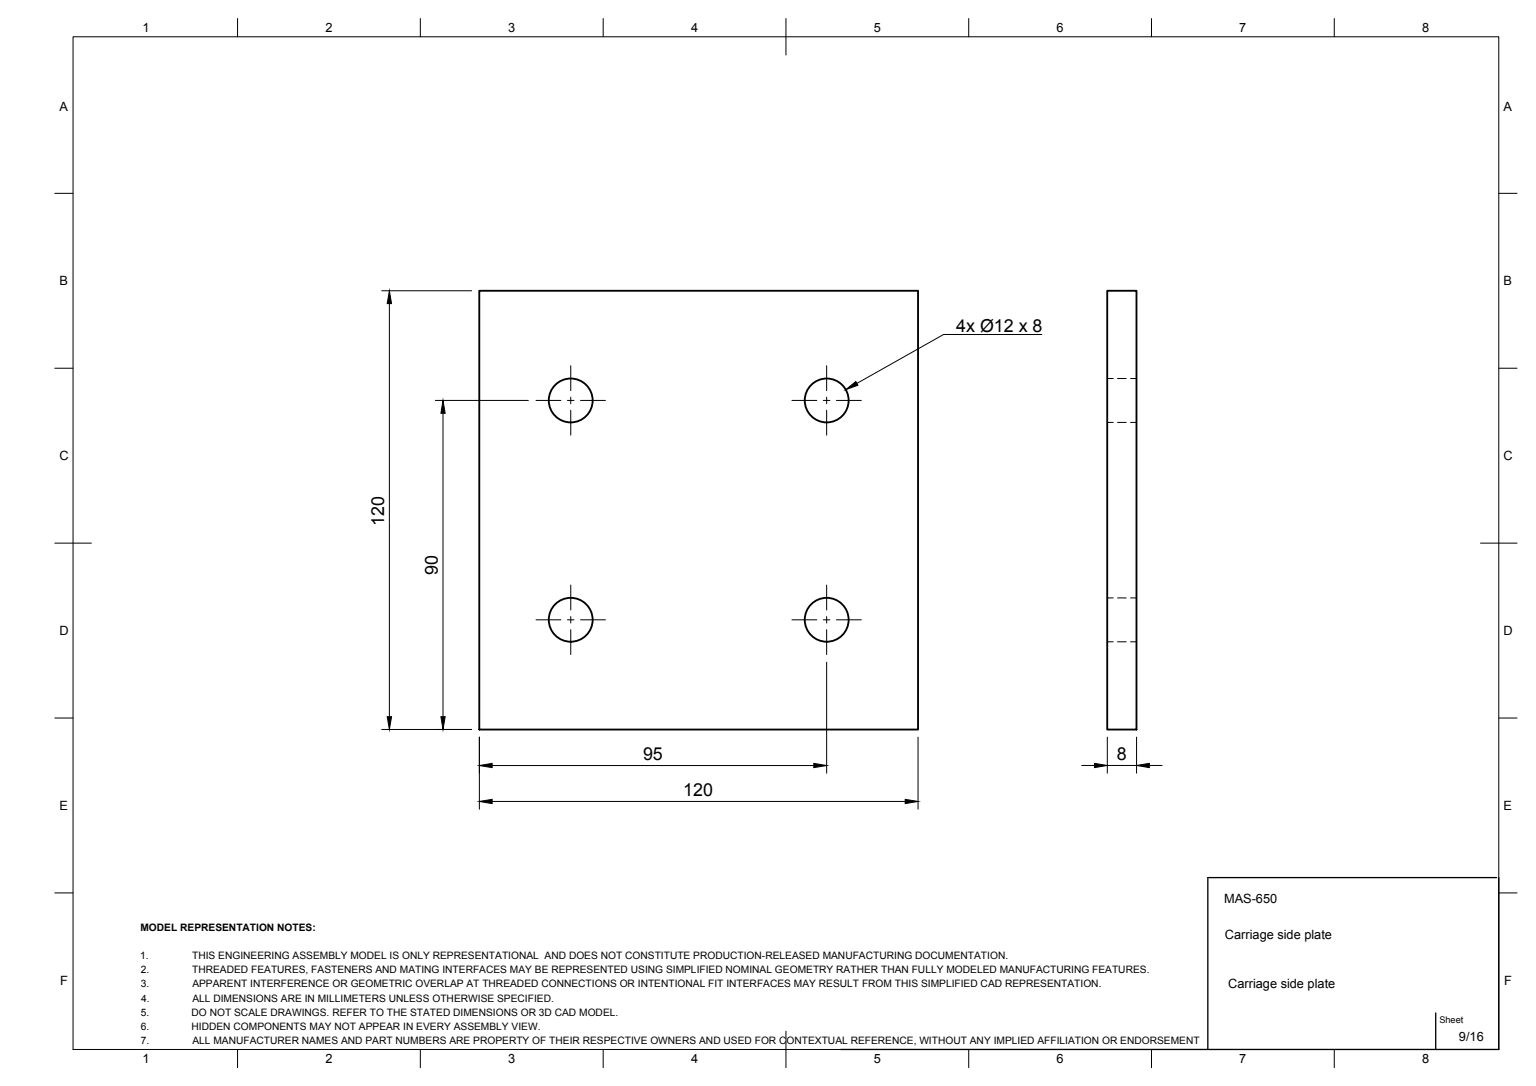
ISO-10303-21;
HEADER;
/* Generated by software containing ST-Developer
 * from STEP Tools, Inc. (www.steptools.com) 
 */

FILE_DESCRIPTION(
/* description */ ('Independent manual traversing gantry with native reusable aluminum pr
ofiles,180mm captured carriage travel, four bronze-bushed rollers, lin
ked ideal rolling motion, bonded acetal lateral guides, positive welde
d end stops and fully retained axle stacks. Editable native profile cu
t lengths220/400mm. Tool attachments viaM6 bridge-plate taps; mounted 
tool outside assembly. Welds, anchors, adhesives, fits, traction, load
/speed/structural/life ratings unassigned.'),
/* implementation_level */ '2;1');

FILE_NAME(
/* name */ 'Carriage side plate.step',
/* time_stamp */ '2026-11-09T20:04:38-08:00',
/* author */ (''),
/* organization */ (''),
/* preprocessor_version */ 'ST-DEVELOPER v20.2',
/* originating_system */ 'Autodesk Translation Framework v15.17.0.0',
/* authorisation */ '');

FILE_SCHEMA (('AUTOMOTIVE_DESIGN { 1 0 10303 214 3 1 1 }'));
ENDSEC;

DATA;
#10=MECHANICAL_DESIGN_GEOMETRIC_PRESENTATION_REPRESENTATION('',(#477),#13231);
#445=SHAPE_REPRESENTATION_RELATIONSHIP('SRR','None',#13334,#461);
#461=ADVANCED_BREP_SHAPE_REPRESENTATION('',(#493),#13221);
#477=STYLED_ITEM('',(#13423),#493);
#493=MANIFOLD_SOLID_BREP('Body1',#4157);
#523=FACE_BOUND('',#947,.T.);
#524=FACE_BOUND('',#948,.T.);
#525=FACE_BOUND('',#949,.T.);
#526=FACE_BOUND('',#950,.T.);
#527=FACE_BOUND('',#953,.T.);
#528=FACE_BOUND('',#954,.T.);
#529=FACE_BOUND('',#955,.T.);
#530=FACE_BOUND('',#956,.T.);
#596=PLANE('',#4480);
#597=PLANE('',#4481);
#598=PLANE('',#4482);
#599=PLANE('',#4483);
#600=PLANE('',#4484);
#601=PLANE('',#4485);
#701=FACE_OUTER_BOUND('',#942,.T.);
#702=FACE_OUTER_BOUND('',#943,.T.);
#703=FACE_OUTER_BOUND('',#944,.T.);
#704=FACE_OUTER_BOUND('',#945,.T.);
#705=FACE_OUTER_BOUND('',#946,.T.);
#706=FACE_OUTER_BOUND('',#951,.T.);
#707=FACE_OUTER_BOUND('',#952,.T.);
#708=FACE_OUTER_BOUND('',#957,.T.);
#709=FACE_OUTER_BOUND('',#958,.T.);
#710=FACE_OUTER_BOUND('',#959,.T.);
#942=EDGE_LOOP('',(#3018,#3019,#3020,#3021));
#943=EDGE_LOOP('',(#3022,#3023,#3024,#3025));
#944=EDGE_LOOP('',(#3026,#3027,#3028,#3029));
#945=EDGE_LOOP('',(#3030,#3031,#3032,#3033));
#946=EDGE_LOOP('',(#3034,#3035,#3036,#3037));
#947=EDGE_LOOP('',(#3038));
#948=EDGE_LOOP('',(#3039));
#949=EDGE_LOOP('',(#3040));
#950=EDGE_LOOP('',(#3041));
#951=EDGE_LOOP('',(#3042,#3043,#3044,#3045));
#952=EDGE_LOOP('',(#3046,#3047,#3048,#3049));
#953=EDGE_LOOP('',(#3050));
#954=EDGE_LOOP('',(#3051));
#955=EDGE_LOOP('',(#3052));
#956=EDGE_LOOP('',(#3053));
#957=EDGE_LOOP('',(#3054,#3055,#3056,#3057));
#958=EDGE_LOOP('',(#3058,#3059,#3060,#3061));
#959=EDGE_LOOP('',(#3062,#3063,#3064,#3065));
#1244=LINE('',#6139,#1506);
#1245=LINE('',#6145,#1507);
#1246=LINE('',#6151,#1508);
#1247=LINE('',#6157,#1509);
#1248=LINE('',#6162,#1510);
#1249=LINE('',#6164,#1511);
#1250=LINE('',#6166,#1512);
#1251=LINE('',#6167,#1513);
#1252=LINE('',#6170,#1514);
#1253=LINE('',#6172,#1515);
#1254=LINE('',#6173,#1516);
#1255=LINE('',#6176,#1517);
#1256=LINE('',#6178,#1518);
#1257=LINE('',#6179,#1519);
#1258=LINE('',#6181,#1520);
#1259=LINE('',#6182,#1521);
#1506=VECTOR('',#5107,6.);
#1507=VECTOR('',#5114,6.);
#1508=VECTOR('',#5121,6.);
#1509=VECTOR('',#5128,6.);
#1510=VECTOR('',#5133,10.);
#1511=VECTOR('',#5134,10.);
#1512=VECTOR('',#5135,10.);
#1513=VECTOR('',#5136,10.);
#1514=VECTOR('',#5139,10.);
#1515=VECTOR('',#5140,10.);
#1516=VECTOR('',#5141,10.);
#1517=VECTOR('',#5144,10.);
#1518=VECTOR('',#5145,10.);
#1519=VECTOR('',#5146,10.);
#1520=VECTOR('',#5149,10.);
#1521=VECTOR('',#5150,10.);
#1696=CIRCLE('',#4469,6.);
#1697=CIRCLE('',#4470,6.);
#1698=CIRCLE('',#4472,6.);
#1699=CIRCLE('',#4473,6.);
#1700=CIRCLE('',#4475,6.);
#1701=CIRCLE('',#4476,6.);
#1702=CIRCLE('',#4478,6.);
#1703=CIRCLE('',#4479,6.);
#1864=VERTEX_POINT('',#6136);
#1865=VERTEX_POINT('',#6138);
#1866=VERTEX_POINT('',#6142);
#1867=VERTEX_POINT('',#6144);
#1868=VERTEX_POINT('',#6148);
#1869=VERTEX_POINT('',#6150);
#1870=VERTEX_POINT('',#6154);
#1871=VERTEX_POINT('',#6156);
#1872=VERTEX_POINT('',#6160);
#1873=VERTEX_POINT('',#6161);
#1874=VERTEX_POINT('',#6163);
#1875=VERTEX_POINT('',#6165);
#1876=VERTEX_POINT('',#6169);
#1877=VERTEX_POINT('',#6171);
#1878=VERTEX_POINT('',#6175);
#1879=VERTEX_POINT('',#6177);
#2292=EDGE_CURVE('',#1864,#1864,#1696,.T.);
#2293=EDGE_CURVE('',#1864,#1865,#1244,.T.);
#2294=EDGE_CURVE('',#1865,#1865,#1697,.T.);
#2295=EDGE_CURVE('',#1866,#1866,#1698,.T.);
#2296=EDGE_CURVE('',#1866,#1867,#1245,.T.);
#2297=EDGE_CURVE('',#1867,#1867,#1699,.T.);
#2298=EDGE_CURVE('',#1868,#1868,#1700,.T.);
#2299=EDGE_CURVE('',#1868,#1869,#1246,.T.);
#2300=EDGE_CURVE('',#1869,#1869,#1701,.T.);
#2301=EDGE_CURVE('',#1870,#1870,#1702,.T.);
#2302=EDGE_CURVE('',#1870,#1871,#1247,.T.);
#2303=EDGE_CURVE('',#1871,#1871,#1703,.T.);
#2304=EDGE_CURVE('',#1872,#1873,#1248,.T.);
#2305=EDGE_CURVE('',#1873,#1874,#1249,.T.);
#2306=EDGE_CURVE('',#1875,#1874,#1250,.T.);
#2307=EDGE_CURVE('',#1872,#1875,#1251,.T.);
#2308=EDGE_CURVE('',#1876,#1872,#1252,.T.);
#2309=EDGE_CURVE('',#1877,#1875,#1253,.T.);
#2310=EDGE_CURVE('',#1876,#1877,#1254,.T.);
#2311=EDGE_CURVE('',#1878,#1876,#1255,.T.);
#2312=EDGE_CURVE('',#1879,#1877,#1256,.T.);
#2313=EDGE_CURVE('',#1878,#1879,#1257,.T.);
#2314=EDGE_CURVE('',#1873,#1878,#1258,.T.);
#2315=EDGE_CURVE('',#1874,#1879,#1259,.T.);
#3018=ORIENTED_EDGE('',*,*,#2292,.F.);
#3019=ORIENTED_EDGE('',*,*,#2293,.T.);
#3020=ORIENTED_EDGE('',*,*,#2294,.F.);
#3021=ORIENTED_EDGE('',*,*,#2293,.F.);
#3022=ORIENTED_EDGE('',*,*,#2295,.F.);
#3023=ORIENTED_EDGE('',*,*,#2296,.T.);
#3024=ORIENTED_EDGE('',*,*,#2297,.F.);
#3025=ORIENTED_EDGE('',*,*,#2296,.F.);
#3026=ORIENTED_EDGE('',*,*,#2298,.F.);
#3027=ORIENTED_EDGE('',*,*,#2299,.T.);
#3028=ORIENTED_EDGE('',*,*,#2300,.F.);
#3029=ORIENTED_EDGE('',*,*,#2299,.F.);
#3030=ORIENTED_EDGE('',*,*,#2301,.F.);
#3031=ORIENTED_EDGE('',*,*,#2302,.T.);
#3032=ORIENTED_EDGE('',*,*,#2303,.F.);
#3033=ORIENTED_EDGE('',*,*,#2302,.F.);
#3034=ORIENTED_EDGE('',*,*,#2304,.T.);
#3035=ORIENTED_EDGE('',*,*,#2305,.T.);
#3036=ORIENTED_EDGE('',*,*,#2306,.F.);
#3037=ORIENTED_EDGE('',*,*,#2307,.F.);
#3038=ORIENTED_EDGE('',*,*,#2292,.T.);
#3039=ORIENTED_EDGE('',*,*,#2295,.T.);
#3040=ORIENTED_EDGE('',*,*,#2298,.T.);
#3041=ORIENTED_EDGE('',*,*,#2301,.T.);
#3042=ORIENTED_EDGE('',*,*,#2308,.T.);
#3043=ORIENTED_EDGE('',*,*,#2307,.T.);
#3044=ORIENTED_EDGE('',*,*,#2309,.F.);
#3045=ORIENTED_EDGE('',*,*,#2310,.F.);
#3046=ORIENTED_EDGE('',*,*,#2311,.T.);
#3047=ORIENTED_EDGE('',*,*,#2310,.T.);
#3048=ORIENTED_EDGE('',*,*,#2312,.F.);
#3049=ORIENTED_EDGE('',*,*,#2313,.F.);
#3050=ORIENTED_EDGE('',*,*,#2294,.T.);
#3051=ORIENTED_EDGE('',*,*,#2297,.T.);
#3052=ORIENTED_EDGE('',*,*,#2300,.T.);
#3053=ORIENTED_EDGE('',*,*,#2303,.T.);
#3054=ORIENTED_EDGE('',*,*,#2314,.T.);
#3055=ORIENTED_EDGE('',*,*,#2313,.T.);
#3056=ORIENTED_EDGE('',*,*,#2315,.F.);
#3057=ORIENTED_EDGE('',*,*,#2305,.F.);
#3058=ORIENTED_EDGE('',*,*,#2315,.T.);
#3059=ORIENTED_EDGE('',*,*,#2312,.T.);
#3060=ORIENTED_EDGE('',*,*,#2309,.T.);
#3061=ORIENTED_EDGE('',*,*,#2306,.T.);
#3062=ORIENTED_EDGE('',*,*,#2314,.F.);
#3063=ORIENTED_EDGE('',*,*,#2304,.F.);
#3064=ORIENTED_EDGE('',*,*,#2308,.F.);
#3065=ORIENTED_EDGE('',*,*,#2311,.F.);
#3822=CYLINDRICAL_SURFACE('',#4468,6.);
#3823=CYLINDRICAL_SURFACE('',#4471,6.);
#3824=CYLINDRICAL_SURFACE('',#4474,6.);
#3825=CYLINDRICAL_SURFACE('',#4477,6.);
#3998=ADVANCED_FACE('',(#701),#3822,.F.);
#3999=ADVANCED_FACE('',(#702),#3823,.F.);
#4000=ADVANCED_FACE('',(#703),#3824,.F.);
#4001=ADVANCED_FACE('',(#704),#3825,.F.);
#4002=ADVANCED_FACE('',(#705,#523,#524,#525,#526),#596,.T.);
#4003=ADVANCED_FACE('',(#706),#597,.T.);
#4004=ADVANCED_FACE('',(#707,#527,#528,#529,#530),#598,.T.);
#4005=ADVANCED_FACE('',(#708),#599,.T.);
#4006=ADVANCED_FACE('',(#709),#600,.T.);
#4007=ADVANCED_FACE('',(#710),#601,.F.);
#4157=CLOSED_SHELL('',(#3998,#3999,#4000,#4001,#4002,#4003,#4004,#4005,
#4006,#4007));
#4467=AXIS2_PLACEMENT_3D('',#6134,#5101,#5102);
#4468=AXIS2_PLACEMENT_3D('',#6135,#5103,#5104);
#4469=AXIS2_PLACEMENT_3D('',#6137,#5105,#5106);
#4470=AXIS2_PLACEMENT_3D('',#6140,#5108,#5109);
#4471=AXIS2_PLACEMENT_3D('',#6141,#5110,#5111);
#4472=AXIS2_PLACEMENT_3D('',#6143,#5112,#5113);
#4473=AXIS2_PLACEMENT_3D('',#6146,#5115,#5116);
#4474=AXIS2_PLACEMENT_3D('',#6147,#5117,#5118);
#4475=AXIS2_PLACEMENT_3D('',#6149,#5119,#5120);
#4476=AXIS2_PLACEMENT_3D('',#6152,#5122,#5123);
#4477=AXIS2_PLACEMENT_3D('',#6153,#5124,#5125);
#4478=AXIS2_PLACEMENT_3D('',#6155,#5126,#5127);
#4479=AXIS2_PLACEMENT_3D('',#6158,#5129,#5130);
#4480=AXIS2_PLACEMENT_3D('',#6159,#5131,#5132);
#4481=AXIS2_PLACEMENT_3D('',#6168,#5137,#5138);
#4482=AXIS2_PLACEMENT_3D('',#6174,#5142,#5143);
#4483=AXIS2_PLACEMENT_3D('',#6180,#5147,#5148);
#4484=AXIS2_PLACEMENT_3D('',#6183,#5151,#5152);
#4485=AXIS2_PLACEMENT_3D('',#6184,#5153,#5154);
#5101=DIRECTION('axis',(0.,0.,1.));
#5102=DIRECTION('refdir',(1.,0.,0.));
#5103=DIRECTION('center_axis',(0.,-1.,0.));
#5104=DIRECTION('ref_axis',(0.,0.,1.));
#5105=DIRECTION('center_axis',(0.,-1.,0.));
#5106=DIRECTION('ref_axis',(0.,0.,1.));
#5107=DIRECTION('',(0.,-1.,0.));
#5108=DIRECTION('center_axis',(0.,1.,0.));
#5109=DIRECTION('ref_axis',(0.,0.,1.));
#5110=DIRECTION('center_axis',(0.,-1.,0.));
#5111=DIRECTION('ref_axis',(0.,0.,1.));
#5112=DIRECTION('center_axis',(0.,-1.,0.));
#5113=DIRECTION('ref_axis',(0.,0.,1.));
#5114=DIRECTION('',(0.,-1.,0.));
#5115=DIRECTION('center_axis',(0.,1.,0.));
#5116=DIRECTION('ref_axis',(0.,0.,1.));
#5117=DIRECTION('center_axis',(0.,-1.,0.));
#5118=DIRECTION('ref_axis',(0.,0.,1.));
#5119=DIRECTION('center_axis',(0.,-1.,0.));
#5120=DIRECTION('ref_axis',(0.,0.,1.));
#5121=DIRECTION('',(0.,-1.,0.));
#5122=DIRECTION('center_axis',(0.,1.,0.));
#5123=DIRECTION('ref_axis',(0.,0.,1.));
#5124=DIRECTION('center_axis',(0.,-1.,0.));
#5125=DIRECTION('ref_axis',(0.,0.,1.));
#5126=DIRECTION('center_axis',(0.,-1.,0.));
#5127=DIRECTION('ref_axis',(0.,0.,1.));
#5128=DIRECTION('',(0.,-1.,0.));
#5129=DIRECTION('center_axis',(0.,1.,0.));
#5130=DIRECTION('ref_axis',(0.,0.,1.));
#5131=DIRECTION('center_axis',(0.,1.,0.));
#5132=DIRECTION('ref_axis',(-1.,0.,0.));
#5133=DIRECTION('',(-1.,0.,0.));
#5134=DIRECTION('',(0.,0.,1.));
#5135=DIRECTION('',(-1.,0.,0.));
#5136=DIRECTION('',(0.,0.,1.));
#5137=DIRECTION('center_axis',(1.,0.,0.));
#5138=DIRECTION('ref_axis',(0.,1.,0.));
#5139=DIRECTION('',(0.,1.,0.));
#5140=DIRECTION('',(0.,1.,0.));
#5141=DIRECTION('',(0.,0.,1.));
#5142=DIRECTION('center_axis',(0.,-1.,0.));
#5143=DIRECTION('ref_axis',(1.,0.,0.));
#5144=DIRECTION('',(1.,0.,0.));
#5145=DIRECTION('',(1.,0.,0.));
#5146=DIRECTION('',(0.,0.,1.));
#5147=DIRECTION('center_axis',(-1.,0.,0.));
#5148=DIRECTION('ref_axis',(0.,-1.,0.));
#5149=DIRECTION('',(0.,-1.,0.));
#5150=DIRECTION('',(0.,-1.,0.));
#5151=DIRECTION('center_axis',(0.,0.,1.));
#5152=DIRECTION('ref_axis',(1.,0.,0.));
#5153=DIRECTION('center_axis',(0.,0.,1.));
#5154=DIRECTION('ref_axis',(1.,0.,0.));
#6134=CARTESIAN_POINT('',(0.,0.,0.));
#6135=CARTESIAN_POINT('Origin',(30.,0.,225.));
#6136=CARTESIAN_POINT('',(30.,4.,219.));
#6137=CARTESIAN_POINT('Origin',(30.,4.,225.));
#6138=CARTESIAN_POINT('',(30.,-4.,219.));
#6139=CARTESIAN_POINT('',(30.,0.,219.));
#6140=CARTESIAN_POINT('Origin',(30.,-4.,225.));
#6141=CARTESIAN_POINT('Origin',(-30.,0.,225.));
#6142=CARTESIAN_POINT('',(-30.,4.,219.));
#6143=CARTESIAN_POINT('Origin',(-30.,4.,225.));
#6144=CARTESIAN_POINT('',(-30.,-4.,219.));
#6145=CARTESIAN_POINT('',(-30.,0.,219.));
#6146=CARTESIAN_POINT('Origin',(-30.,-4.,225.));
#6147=CARTESIAN_POINT('Origin',(-30.,0.,295.));
#6148=CARTESIAN_POINT('',(-30.,4.,289.));
#6149=CARTESIAN_POINT('Origin',(-30.,4.,295.));
#6150=CARTESIAN_POINT('',(-30.,-4.,289.));
#6151=CARTESIAN_POINT('',(-30.,0.,289.));
#6152=CARTESIAN_POINT('Origin',(-30.,-4.,295.));
#6153=CARTESIAN_POINT('Origin',(30.,0.,295.));
#6154=CARTESIAN_POINT('',(30.,4.,289.));
#6155=CARTESIAN_POINT('Origin',(30.,4.,295.));
#6156=CARTESIAN_POINT('',(30.,-4.,289.));
#6157=CARTESIAN_POINT('',(30.,0.,289.));
#6158=CARTESIAN_POINT('Origin',(30.,-4.,295.));
#6159=CARTESIAN_POINT('Origin',(60.,4.,200.));
#6160=CARTESIAN_POINT('',(60.,4.,200.));
#6161=CARTESIAN_POINT('',(-60.,4.,200.));
#6162=CARTESIAN_POINT('',(60.,4.,200.));
#6163=CARTESIAN_POINT('',(-60.,4.,320.));
#6164=CARTESIAN_POINT('',(-60.,4.,200.));
#6165=CARTESIAN_POINT('',(60.,4.,320.));
#6166=CARTESIAN_POINT('',(60.,4.,320.));
#6167=CARTESIAN_POINT('',(60.,4.,200.));
#6168=CARTESIAN_POINT('Origin',(60.,-4.,200.));
#6169=CARTESIAN_POINT('',(60.,-4.,200.));
#6170=CARTESIAN_POINT('',(60.,-4.,200.));
#6171=CARTESIAN_POINT('',(60.,-4.,320.));
#6172=CARTESIAN_POINT('',(60.,-4.,320.));
#6173=CARTESIAN_POINT('',(60.,-4.,200.));
#6174=CARTESIAN_POINT('Origin',(-60.,-4.,200.));
#6175=CARTESIAN_POINT('',(-60.,-4.,200.));
#6176=CARTESIAN_POINT('',(-60.,-4.,200.));
#6177=CARTESIAN_POINT('',(-60.,-4.,320.));
#6178=CARTESIAN_POINT('',(-60.,-4.,320.));
#6179=CARTESIAN_POINT('',(-60.,-4.,200.));
#6180=CARTESIAN_POINT('Origin',(-60.,4.,200.));
#6181=CARTESIAN_POINT('',(-60.,4.,200.));
#6182=CARTESIAN_POINT('',(-60.,4.,320.));
#6183=CARTESIAN_POINT('Origin',(0.,0.,320.));
#6184=CARTESIAN_POINT('Origin',(0.,0.,200.));
#13203=UNCERTAINTY_MEASURE_WITH_UNIT(LENGTH_MEASURE(0.01),#13232,
'DISTANCE_ACCURACY_VALUE',
'Maximum model space distance between geometric entities at asserted c
onnectivities');
#13213=UNCERTAINTY_MEASURE_WITH_UNIT(LENGTH_MEASURE(0.01),#13232,
'DISTANCE_ACCURACY_VALUE',
'Maximum model space distance between geometric entities at asserted c
onnectivities');
#13221=(
GEOMETRIC_REPRESENTATION_CONTEXT(3)
GLOBAL_UNCERTAINTY_ASSIGNED_CONTEXT((#13203))
GLOBAL_UNIT_ASSIGNED_CONTEXT((#13232,#13234,#13235))
REPRESENTATION_CONTEXT('','3D')
);
#13231=(
GEOMETRIC_REPRESENTATION_CONTEXT(3)
GLOBAL_UNCERTAINTY_ASSIGNED_CONTEXT((#13213))
GLOBAL_UNIT_ASSIGNED_CONTEXT((#13232,#13234,#13235))
REPRESENTATION_CONTEXT('','3D')
);
#13232=(
LENGTH_UNIT()
NAMED_UNIT(*)
SI_UNIT(.MILLI.,.METRE.)
);
#13234=(
NAMED_UNIT(*)
PLANE_ANGLE_UNIT()
SI_UNIT($,.RADIAN.)
);
#13235=(
NAMED_UNIT(*)
SI_UNIT($,.STERADIAN.)
SOLID_ANGLE_UNIT()
);
#13243=SHAPE_DEFINITION_REPRESENTATION(#13260,#13334);
#13260=PRODUCT_DEFINITION_SHAPE('',$,#13352);
#13334=SHAPE_REPRESENTATION('',(#4467),#13221);
#13344=PRODUCT_DEFINITION_CONTEXT('part definition',#13397,'design');
#13352=PRODUCT_DEFINITION('Carriage side plate','Carriage side plate',#13369,
#13344);
#13369=PRODUCT_DEFINITION_FORMATION('',$,#13406);
#13397=APPLICATION_CONTEXT(
'Core Data for Automotive Mechanical Design Process');
#13398=PRODUCT_CONTEXT('part definition',#13397,'mechanical');
#13406=PRODUCT('Carriage side plate','Carriage side plate',$,(#13398));
#13423=PRESENTATION_STYLE_ASSIGNMENT((#13437));
#13437=SURFACE_STYLE_USAGE(.BOTH.,#13451);
#13451=SURFACE_SIDE_STYLE('',(#13465));
#13465=SURFACE_STYLE_FILL_AREA(#13479);
#13479=FILL_AREA_STYLE('Light blue',(#13493));
#13493=FILL_AREA_STYLE_COLOUR('Light blue',#13507);
#13507=COLOUR_RGB('Light blue',0.662745098039216,0.831372549019608,0.949019607843137);
ENDSEC;
END-ISO-10303-21;
